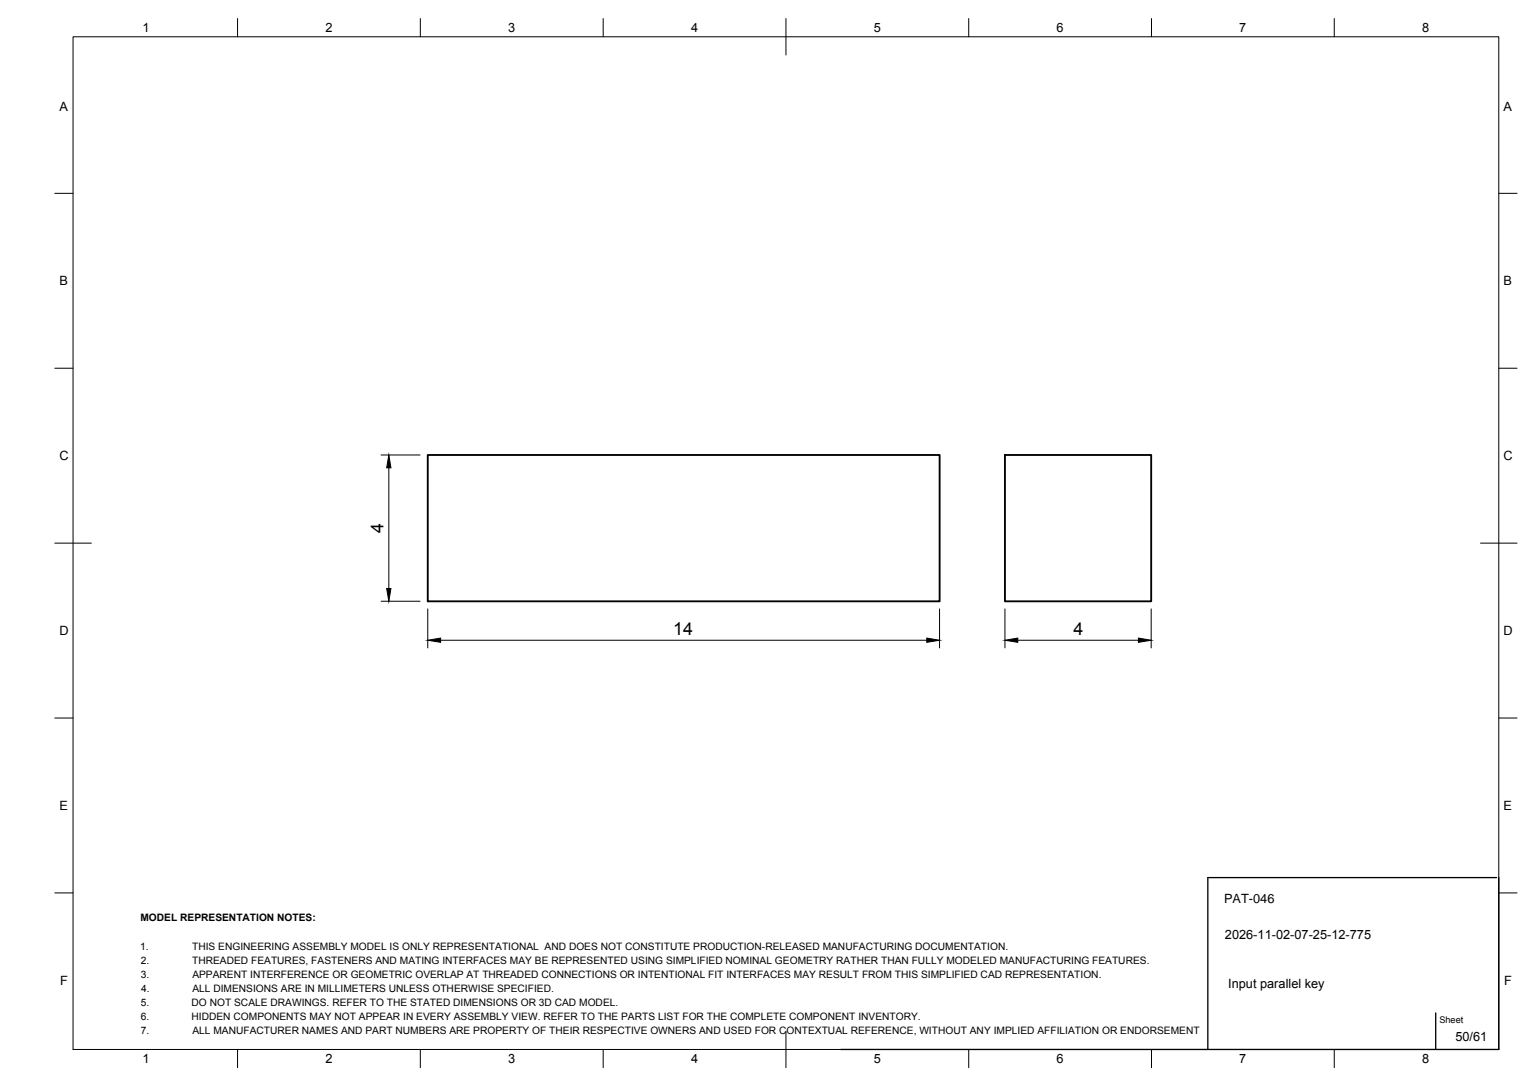
ISO-10303-21;
HEADER;
/* Generated by software containing ST-Developer
 * from STEP Tools, Inc. (www.steptools.com) 
 */

FILE_DESCRIPTION(
/* description */ ('Gear mesh backlash fixture'),
/* implementation_level */ '2;1');

FILE_NAME(
/* name */ 'Input parallel key.step',
/* time_stamp */ '2026-10-28T03:26:00-07:00',
/* author */ (''),
/* organization */ (''),
/* preprocessor_version */ 'ST-DEVELOPER v20.2',
/* originating_system */ 'Autodesk Translation Framework v15.17.0.0',
/* authorisation */ '');

FILE_SCHEMA (('AUTOMOTIVE_DESIGN { 1 0 10303 214 3 1 1 }'));
ENDSEC;

DATA;
#10=MECHANICAL_DESIGN_GEOMETRIC_PRESENTATION_REPRESENTATION('',(#1069),#57900);
#954=SHAPE_REPRESENTATION_RELATIONSHIP('SRR','None',#58154,#1004);
#1004=ADVANCED_BREP_SHAPE_REPRESENTATION('',(#1132),#57887);
#1069=STYLED_ITEM('',(#58465),#1132);
#1132=MANIFOLD_SOLID_BREP('Body1',#13631);
#1570=PLANE('',#15113);
#1571=PLANE('',#15114);
#1572=PLANE('',#15115);
#1573=PLANE('',#15116);
#1574=PLANE('',#15117);
#1575=PLANE('',#15118);
#2129=FACE_OUTER_BOUND('',#3057,.T.);
#2130=FACE_OUTER_BOUND('',#3058,.T.);
#2131=FACE_OUTER_BOUND('',#3059,.T.);
#2132=FACE_OUTER_BOUND('',#3060,.T.);
#2133=FACE_OUTER_BOUND('',#3061,.T.);
#2134=FACE_OUTER_BOUND('',#3062,.T.);
#3057=EDGE_LOOP('',(#10813,#10814,#10815,#10816));
#3058=EDGE_LOOP('',(#10817,#10818,#10819,#10820));
#3059=EDGE_LOOP('',(#10821,#10822,#10823,#10824));
#3060=EDGE_LOOP('',(#10825,#10826,#10827,#10828));
#3061=EDGE_LOOP('',(#10829,#10830,#10831,#10832));
#3062=EDGE_LOOP('',(#10833,#10834,#10835,#10836));
#3906=LINE('',#22185,#4795);
#3907=LINE('',#22187,#4796);
#3908=LINE('',#22189,#4797);
#3909=LINE('',#22190,#4798);
#3910=LINE('',#22193,#4799);
#3911=LINE('',#22195,#4800);
#3912=LINE('',#22196,#4801);
#3913=LINE('',#22199,#4802);
#3914=LINE('',#22201,#4803);
#3915=LINE('',#22202,#4804);
#3916=LINE('',#22204,#4805);
#3917=LINE('',#22205,#4806);
#4795=VECTOR('',#17911,1.);
#4796=VECTOR('',#17912,1.);
#4797=VECTOR('',#17913,1.);
#4798=VECTOR('',#17914,1.);
#4799=VECTOR('',#17917,1.);
#4800=VECTOR('',#17918,1.);
#4801=VECTOR('',#17919,1.);
#4802=VECTOR('',#17922,1.);
#4803=VECTOR('',#17923,1.);
#4804=VECTOR('',#17924,1.);
#4805=VECTOR('',#17927,1.);
#4806=VECTOR('',#17928,1.);
#6436=VERTEX_POINT('',#22183);
#6437=VERTEX_POINT('',#22184);
#6438=VERTEX_POINT('',#22186);
#6439=VERTEX_POINT('',#22188);
#6440=VERTEX_POINT('',#22192);
#6441=VERTEX_POINT('',#22194);
#6442=VERTEX_POINT('',#22198);
#6443=VERTEX_POINT('',#22200);
#7993=EDGE_CURVE('',#6436,#6437,#3906,.T.);
#7994=EDGE_CURVE('',#6436,#6438,#3907,.T.);
#7995=EDGE_CURVE('',#6439,#6438,#3908,.T.);
#7996=EDGE_CURVE('',#6437,#6439,#3909,.T.);
#7997=EDGE_CURVE('',#6437,#6440,#3910,.T.);
#7998=EDGE_CURVE('',#6441,#6439,#3911,.T.);
#7999=EDGE_CURVE('',#6440,#6441,#3912,.T.);
#8000=EDGE_CURVE('',#6440,#6442,#3913,.T.);
#8001=EDGE_CURVE('',#6443,#6441,#3914,.T.);
#8002=EDGE_CURVE('',#6442,#6443,#3915,.T.);
#8003=EDGE_CURVE('',#6442,#6436,#3916,.T.);
#8004=EDGE_CURVE('',#6438,#6443,#3917,.T.);
#10813=ORIENTED_EDGE('',*,*,#7993,.F.);
#10814=ORIENTED_EDGE('',*,*,#7994,.T.);
#10815=ORIENTED_EDGE('',*,*,#7995,.F.);
#10816=ORIENTED_EDGE('',*,*,#7996,.F.);
#10817=ORIENTED_EDGE('',*,*,#7997,.F.);
#10818=ORIENTED_EDGE('',*,*,#7996,.T.);
#10819=ORIENTED_EDGE('',*,*,#7998,.F.);
#10820=ORIENTED_EDGE('',*,*,#7999,.F.);
#10821=ORIENTED_EDGE('',*,*,#8000,.F.);
#10822=ORIENTED_EDGE('',*,*,#7999,.T.);
#10823=ORIENTED_EDGE('',*,*,#8001,.F.);
#10824=ORIENTED_EDGE('',*,*,#8002,.F.);
#10825=ORIENTED_EDGE('',*,*,#8003,.F.);
#10826=ORIENTED_EDGE('',*,*,#8002,.T.);
#10827=ORIENTED_EDGE('',*,*,#8004,.F.);
#10828=ORIENTED_EDGE('',*,*,#7994,.F.);
#10829=ORIENTED_EDGE('',*,*,#8004,.T.);
#10830=ORIENTED_EDGE('',*,*,#8001,.T.);
#10831=ORIENTED_EDGE('',*,*,#7998,.T.);
#10832=ORIENTED_EDGE('',*,*,#7995,.T.);
#10833=ORIENTED_EDGE('',*,*,#8003,.T.);
#10834=ORIENTED_EDGE('',*,*,#7993,.T.);
#10835=ORIENTED_EDGE('',*,*,#7997,.T.);
#10836=ORIENTED_EDGE('',*,*,#8000,.T.);
#13246=ADVANCED_FACE('',(#2129),#1570,.T.);
#13247=ADVANCED_FACE('',(#2130),#1571,.T.);
#13248=ADVANCED_FACE('',(#2131),#1572,.T.);
#13249=ADVANCED_FACE('',(#2132),#1573,.T.);
#13250=ADVANCED_FACE('',(#2133),#1574,.T.);
#13251=ADVANCED_FACE('',(#2134),#1575,.F.);
#13631=CLOSED_SHELL('',(#13246,#13247,#13248,#13249,#13250,#13251));
#15112=AXIS2_PLACEMENT_3D('',#22181,#17907,#17908);
#15113=AXIS2_PLACEMENT_3D('',#22182,#17909,#17910);
#15114=AXIS2_PLACEMENT_3D('',#22191,#17915,#17916);
#15115=AXIS2_PLACEMENT_3D('',#22197,#17920,#17921);
#15116=AXIS2_PLACEMENT_3D('',#22203,#17925,#17926);
#15117=AXIS2_PLACEMENT_3D('',#22206,#17929,#17930);
#15118=AXIS2_PLACEMENT_3D('',#22207,#17931,#17932);
#17907=DIRECTION('axis',(0.,0.,1.));
#17908=DIRECTION('refdir',(1.,0.,0.));
#17909=DIRECTION('center_axis',(0.,-1.,0.));
#17910=DIRECTION('ref_axis',(1.,0.,0.));
#17911=DIRECTION('',(-1.,0.,0.));
#17912=DIRECTION('',(0.,0.,1.));
#17913=DIRECTION('',(1.,0.,0.));
#17914=DIRECTION('',(0.,0.,1.));
#17915=DIRECTION('center_axis',(-1.,0.,0.));
#17916=DIRECTION('ref_axis',(0.,-1.,0.));
#17917=DIRECTION('',(0.,1.,0.));
#17918=DIRECTION('',(0.,-1.,0.));
#17919=DIRECTION('',(0.,0.,1.));
#17920=DIRECTION('center_axis',(0.,1.,0.));
#17921=DIRECTION('ref_axis',(-1.,0.,0.));
#17922=DIRECTION('',(1.,0.,0.));
#17923=DIRECTION('',(-1.,0.,0.));
#17924=DIRECTION('',(0.,0.,1.));
#17925=DIRECTION('center_axis',(1.,0.,0.));
#17926=DIRECTION('ref_axis',(0.,1.,0.));
#17927=DIRECTION('',(0.,-1.,0.));
#17928=DIRECTION('',(0.,1.,0.));
#17929=DIRECTION('center_axis',(0.,0.,1.));
#17930=DIRECTION('ref_axis',(1.,0.,0.));
#17931=DIRECTION('center_axis',(0.,0.,1.));
#17932=DIRECTION('ref_axis',(1.,0.,0.));
#22181=CARTESIAN_POINT('',(0.,0.,0.));
#22182=CARTESIAN_POINT('Origin',(-0.2,0.35,11.8));
#22183=CARTESIAN_POINT('',(0.2,0.35,11.8));
#22184=CARTESIAN_POINT('',(-0.2,0.35,11.8));
#22185=CARTESIAN_POINT('',(0.2,0.35,11.8));
#22186=CARTESIAN_POINT('',(0.2,0.35,13.2));
#22187=CARTESIAN_POINT('',(0.2,0.35,11.8));
#22188=CARTESIAN_POINT('',(-0.2,0.35,13.2));
#22189=CARTESIAN_POINT('',(0.2,0.35,13.2));
#22190=CARTESIAN_POINT('',(-0.2,0.35,11.8));
#22191=CARTESIAN_POINT('Origin',(-0.2,0.75,11.8));
#22192=CARTESIAN_POINT('',(-0.2,0.75,11.8));
#22193=CARTESIAN_POINT('',(-0.2,0.35,11.8));
#22194=CARTESIAN_POINT('',(-0.2,0.75,13.2));
#22195=CARTESIAN_POINT('',(-0.2,0.35,13.2));
#22196=CARTESIAN_POINT('',(-0.2,0.75,11.8));
#22197=CARTESIAN_POINT('Origin',(0.2,0.75,11.8));
#22198=CARTESIAN_POINT('',(0.2,0.75,11.8));
#22199=CARTESIAN_POINT('',(-0.2,0.75,11.8));
#22200=CARTESIAN_POINT('',(0.2,0.75,13.2));
#22201=CARTESIAN_POINT('',(-0.2,0.75,13.2));
#22202=CARTESIAN_POINT('',(0.2,0.75,11.8));
#22203=CARTESIAN_POINT('Origin',(0.2,0.35,11.8));
#22204=CARTESIAN_POINT('',(0.2,0.75,11.8));
#22205=CARTESIAN_POINT('',(0.2,0.75,13.2));
#22206=CARTESIAN_POINT('Origin',(0.,0.55,13.2));
#22207=CARTESIAN_POINT('Origin',(0.,0.55,11.8));
#57828=UNCERTAINTY_MEASURE_WITH_UNIT(LENGTH_MEASURE(0.001),#57901,
'DISTANCE_ACCURACY_VALUE',
'Maximum model space distance between geometric entities at asserted c
onnectivities');
#57841=UNCERTAINTY_MEASURE_WITH_UNIT(LENGTH_MEASURE(0.001),#57901,
'DISTANCE_ACCURACY_VALUE',
'Maximum model space distance between geometric entities at asserted c
onnectivities');
#57887=(
GEOMETRIC_REPRESENTATION_CONTEXT(3)
GLOBAL_UNCERTAINTY_ASSIGNED_CONTEXT((#57828))
GLOBAL_UNIT_ASSIGNED_CONTEXT((#57901,#57903,#57904))
REPRESENTATION_CONTEXT('','3D')
);
#57900=(
GEOMETRIC_REPRESENTATION_CONTEXT(3)
GLOBAL_UNCERTAINTY_ASSIGNED_CONTEXT((#57841))
GLOBAL_UNIT_ASSIGNED_CONTEXT((#57901,#57903,#57904))
REPRESENTATION_CONTEXT('','3D')
);
#57901=(
LENGTH_UNIT()
NAMED_UNIT(*)
SI_UNIT(.CENTI.,.METRE.)
);
#57903=(
NAMED_UNIT(*)
PLANE_ANGLE_UNIT()
SI_UNIT($,.RADIAN.)
);
#57904=(
NAMED_UNIT(*)
SI_UNIT($,.STERADIAN.)
SOLID_ANGLE_UNIT()
);
#57950=SHAPE_DEFINITION_REPRESENTATION(#58021,#58154);
#58021=PRODUCT_DEFINITION_SHAPE('',$,#58213);
#58154=SHAPE_REPRESENTATION('',(#15112),#57887);
#58167=PRODUCT_DEFINITION_CONTEXT('part definition',#58343,'design');
#58213=PRODUCT_DEFINITION('Input parallel key','Input parallel key',#58271,
#58167);
#58271=PRODUCT_DEFINITION_FORMATION('',$,#58390);
#58343=APPLICATION_CONTEXT(
'Core Data for Automotive Mechanical Design Process');
#58344=PRODUCT_CONTEXT('part definition',#58343,'mechanical');
#58390=PRODUCT('Input parallel key','Input parallel key',
'Input parallel key',(#58344));
#58459=COLOUR_RGB('Grey',0.48,0.52,0.57);
#58460=FILL_AREA_STYLE_COLOUR('',#58459);
#58461=FILL_AREA_STYLE('',(#58460));
#58462=SURFACE_STYLE_FILL_AREA(#58461);
#58463=SURFACE_SIDE_STYLE('',(#58462));
#58464=SURFACE_STYLE_USAGE(.BOTH.,#58463);
#58465=PRESENTATION_STYLE_ASSIGNMENT((#58464));
ENDSEC;
END-ISO-10303-21;
